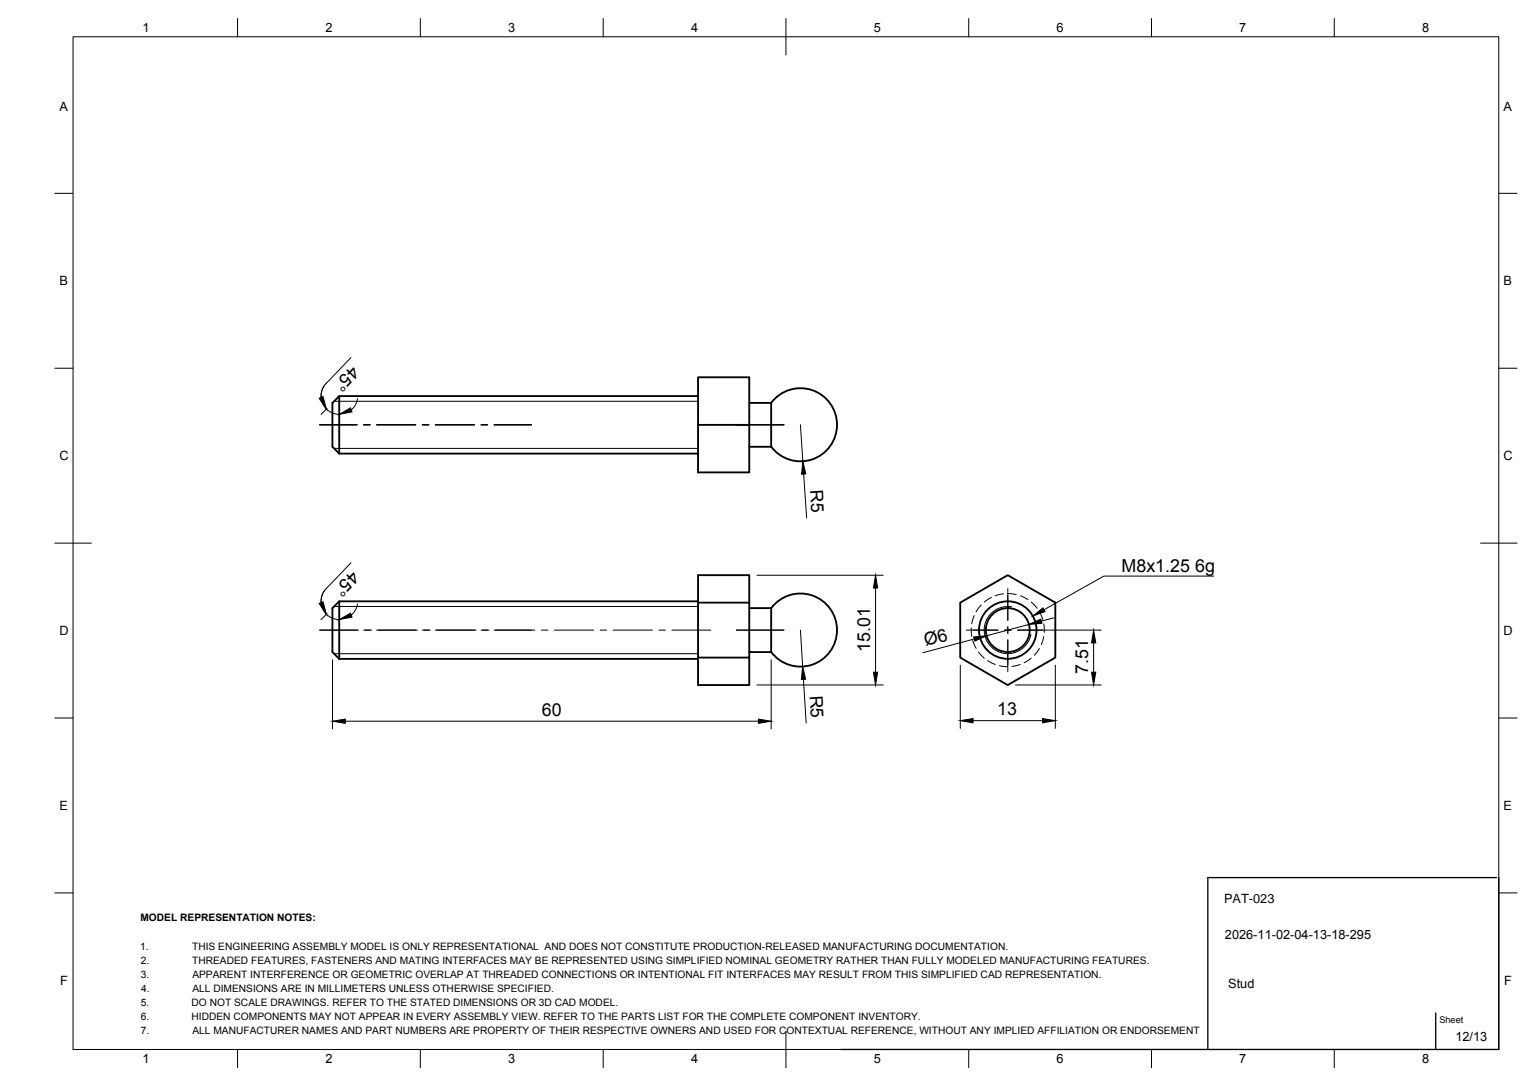
ISO-10303-21;
HEADER;
/* Generated by software containing ST-Developer
 * from STEP Tools, Inc. (www.steptools.com) 
 */

FILE_DESCRIPTION(
/* description */ ('PAT-023'),
/* implementation_level */ '2;1');

FILE_NAME(
/* name */ 'Stud.step',
/* time_stamp */ '2026-10-29T15:47:46-07:00',
/* author */ (''),
/* organization */ (''),
/* preprocessor_version */ 'ST-DEVELOPER v20.2',
/* originating_system */ 'Autodesk Translation Framework v15.17.0.0',
/* authorisation */ '');

FILE_SCHEMA (('AUTOMOTIVE_DESIGN { 1 0 10303 214 3 1 1 }'));
ENDSEC;

DATA;
#10=MECHANICAL_DESIGN_GEOMETRIC_PRESENTATION_REPRESENTATION('',(#89),#3773);
#62=SPHERICAL_SURFACE('',#2421,0.5);
#65=CONICAL_SURFACE('',#2418,0.35,0.78539816339745);
#73=SHAPE_REPRESENTATION_RELATIONSHIP('SRR','None',#3821,#81);
#81=ADVANCED_BREP_SHAPE_REPRESENTATION('',(#97),#3769);
#89=STYLED_ITEM('',(#3953),#97);
#97=MANIFOLD_SOLID_BREP('Body1',#2242);
#110=FACE_BOUND('',#395,.T.);
#111=FACE_BOUND('',#404,.T.);
#154=PLANE('',#2404);
#155=PLANE('',#2406);
#156=PLANE('',#2407);
#157=PLANE('',#2408);
#158=PLANE('',#2409);
#159=PLANE('',#2410);
#160=PLANE('',#2411);
#161=PLANE('',#2415);
#162=PLANE('',#2420);
#265=FACE_OUTER_BOUND('',#394,.T.);
#266=FACE_OUTER_BOUND('',#396,.T.);
#267=FACE_OUTER_BOUND('',#397,.T.);
#268=FACE_OUTER_BOUND('',#398,.T.);
#269=FACE_OUTER_BOUND('',#399,.T.);
#270=FACE_OUTER_BOUND('',#400,.T.);
#271=FACE_OUTER_BOUND('',#401,.T.);
#272=FACE_OUTER_BOUND('',#402,.T.);
#273=FACE_OUTER_BOUND('',#403,.T.);
#274=FACE_OUTER_BOUND('',#405,.T.);
#275=FACE_OUTER_BOUND('',#406,.T.);
#276=FACE_OUTER_BOUND('',#407,.T.);
#277=FACE_OUTER_BOUND('',#408,.T.);
#394=EDGE_LOOP('',(#1735,#1736,#1737,#1738,#1739,#1740));
#395=EDGE_LOOP('',(#1741));
#396=EDGE_LOOP('',(#1742,#1743,#1744,#1745));
#397=EDGE_LOOP('',(#1746,#1747,#1748,#1749));
#398=EDGE_LOOP('',(#1750,#1751,#1752,#1753));
#399=EDGE_LOOP('',(#1754,#1755,#1756,#1757));
#400=EDGE_LOOP('',(#1758,#1759,#1760,#1761));
#401=EDGE_LOOP('',(#1762,#1763,#1764,#1765));
#402=EDGE_LOOP('',(#1766,#1767,#1768,#1769));
#403=EDGE_LOOP('',(#1770,#1771,#1772,#1773,#1774,#1775));
#404=EDGE_LOOP('',(#1776));
#405=EDGE_LOOP('',(#1777,#1778,#1779,#1780));
#406=EDGE_LOOP('',(#1781,#1782,#1783,#1784));
#407=EDGE_LOOP('',(#1785));
#408=EDGE_LOOP('',(#1786,#1787,#1788));
#566=LINE('',#3342,#830);
#567=LINE('',#3344,#831);
#568=LINE('',#3346,#832);
#569=LINE('',#3348,#833);
#570=LINE('',#3350,#834);
#571=LINE('',#3351,#835);
#572=LINE('',#3357,#836);
#573=LINE('',#3358,#837);
#574=LINE('',#3359,#838);
#575=LINE('',#3362,#839);
#576=LINE('',#3363,#840);
#577=LINE('',#3366,#841);
#578=LINE('',#3367,#842);
#579=LINE('',#3370,#843);
#580=LINE('',#3371,#844);
#581=LINE('',#3374,#845);
#582=LINE('',#3375,#846);
#583=LINE('',#3377,#847);
#584=LINE('',#3382,#848);
#585=LINE('',#3388,#849);
#586=LINE('',#3392,#850);
#830=VECTOR('',#2739,1.);
#831=VECTOR('',#2740,1.);
#832=VECTOR('',#2741,1.);
#833=VECTOR('',#2742,1.);
#834=VECTOR('',#2743,1.);
#835=VECTOR('',#2744,1.);
#836=VECTOR('',#2749,1.);
#837=VECTOR('',#2750,1.);
#838=VECTOR('',#2751,1.);
#839=VECTOR('',#2754,1.);
#840=VECTOR('',#2755,1.);
#841=VECTOR('',#2758,1.);
#842=VECTOR('',#2759,1.);
#843=VECTOR('',#2762,1.);
#844=VECTOR('',#2763,1.);
#845=VECTOR('',#2766,1.);
#846=VECTOR('',#2767,1.);
#847=VECTOR('',#2770,1.);
#848=VECTOR('',#2775,0.3);
#849=VECTOR('',#2784,0.4);
#850=VECTOR('',#2789,0.35);
#1013=CIRCLE('',#2405,0.3933);
#1014=CIRCLE('',#2413,0.3);
#1015=CIRCLE('',#2414,0.3);
#1016=CIRCLE('',#2417,0.3933);
#1017=CIRCLE('',#2419,0.3);
#1018=CIRCLE('',#2422,0.5);
#1097=VERTEX_POINT('',#3340);
#1098=VERTEX_POINT('',#3341);
#1099=VERTEX_POINT('',#3343);
#1100=VERTEX_POINT('',#3345);
#1101=VERTEX_POINT('',#3347);
#1102=VERTEX_POINT('',#3349);
#1103=VERTEX_POINT('',#3352);
#1104=VERTEX_POINT('',#3355);
#1105=VERTEX_POINT('',#3356);
#1106=VERTEX_POINT('',#3361);
#1107=VERTEX_POINT('',#3365);
#1108=VERTEX_POINT('',#3369);
#1109=VERTEX_POINT('',#3373);
#1110=VERTEX_POINT('',#3379);
#1111=VERTEX_POINT('',#3381);
#1112=VERTEX_POINT('',#3386);
#1113=VERTEX_POINT('',#3390);
#1114=VERTEX_POINT('',#3395);
#1330=EDGE_CURVE('',#1097,#1098,#566,.T.);
#1331=EDGE_CURVE('',#1098,#1099,#567,.T.);
#1332=EDGE_CURVE('',#1099,#1100,#568,.T.);
#1333=EDGE_CURVE('',#1100,#1101,#569,.T.);
#1334=EDGE_CURVE('',#1101,#1102,#570,.T.);
#1335=EDGE_CURVE('',#1102,#1097,#571,.T.);
#1336=EDGE_CURVE('',#1103,#1103,#1013,.F.);
#1337=EDGE_CURVE('',#1104,#1105,#572,.T.);
#1338=EDGE_CURVE('',#1105,#1097,#573,.T.);
#1339=EDGE_CURVE('',#1104,#1102,#574,.T.);
#1340=EDGE_CURVE('',#1106,#1104,#575,.T.);
#1341=EDGE_CURVE('',#1106,#1101,#576,.T.);
#1342=EDGE_CURVE('',#1107,#1106,#577,.T.);
#1343=EDGE_CURVE('',#1107,#1100,#578,.T.);
#1344=EDGE_CURVE('',#1108,#1107,#579,.T.);
#1345=EDGE_CURVE('',#1108,#1099,#580,.T.);
#1346=EDGE_CURVE('',#1109,#1108,#581,.T.);
#1347=EDGE_CURVE('',#1109,#1098,#582,.T.);
#1348=EDGE_CURVE('',#1105,#1109,#583,.T.);
#1349=EDGE_CURVE('',#1110,#1110,#1014,.T.);
#1350=EDGE_CURVE('',#1110,#1111,#584,.T.);
#1351=EDGE_CURVE('',#1111,#1111,#1015,.T.);
#1352=EDGE_CURVE('',#1112,#1112,#1016,.F.);
#1353=EDGE_CURVE('',#1112,#1103,#585,.T.);
#1354=EDGE_CURVE('',#1113,#1113,#1017,.T.);
#1355=EDGE_CURVE('',#1113,#1112,#586,.T.);
#1356=EDGE_CURVE('',#1111,#1114,#1018,.T.);
#1735=ORIENTED_EDGE('',*,*,#1330,.T.);
#1736=ORIENTED_EDGE('',*,*,#1331,.T.);
#1737=ORIENTED_EDGE('',*,*,#1332,.T.);
#1738=ORIENTED_EDGE('',*,*,#1333,.T.);
#1739=ORIENTED_EDGE('',*,*,#1334,.T.);
#1740=ORIENTED_EDGE('',*,*,#1335,.T.);
#1741=ORIENTED_EDGE('',*,*,#1336,.F.);
#1742=ORIENTED_EDGE('',*,*,#1337,.T.);
#1743=ORIENTED_EDGE('',*,*,#1338,.T.);
#1744=ORIENTED_EDGE('',*,*,#1335,.F.);
#1745=ORIENTED_EDGE('',*,*,#1339,.F.);
#1746=ORIENTED_EDGE('',*,*,#1340,.T.);
#1747=ORIENTED_EDGE('',*,*,#1339,.T.);
#1748=ORIENTED_EDGE('',*,*,#1334,.F.);
#1749=ORIENTED_EDGE('',*,*,#1341,.F.);
#1750=ORIENTED_EDGE('',*,*,#1342,.T.);
#1751=ORIENTED_EDGE('',*,*,#1341,.T.);
#1752=ORIENTED_EDGE('',*,*,#1333,.F.);
#1753=ORIENTED_EDGE('',*,*,#1343,.F.);
#1754=ORIENTED_EDGE('',*,*,#1344,.T.);
#1755=ORIENTED_EDGE('',*,*,#1343,.T.);
#1756=ORIENTED_EDGE('',*,*,#1332,.F.);
#1757=ORIENTED_EDGE('',*,*,#1345,.F.);
#1758=ORIENTED_EDGE('',*,*,#1346,.T.);
#1759=ORIENTED_EDGE('',*,*,#1345,.T.);
#1760=ORIENTED_EDGE('',*,*,#1331,.F.);
#1761=ORIENTED_EDGE('',*,*,#1347,.F.);
#1762=ORIENTED_EDGE('',*,*,#1348,.T.);
#1763=ORIENTED_EDGE('',*,*,#1347,.T.);
#1764=ORIENTED_EDGE('',*,*,#1330,.F.);
#1765=ORIENTED_EDGE('',*,*,#1338,.F.);
#1766=ORIENTED_EDGE('',*,*,#1349,.F.);
#1767=ORIENTED_EDGE('',*,*,#1350,.T.);
#1768=ORIENTED_EDGE('',*,*,#1351,.F.);
#1769=ORIENTED_EDGE('',*,*,#1350,.F.);
#1770=ORIENTED_EDGE('',*,*,#1348,.F.);
#1771=ORIENTED_EDGE('',*,*,#1337,.F.);
#1772=ORIENTED_EDGE('',*,*,#1340,.F.);
#1773=ORIENTED_EDGE('',*,*,#1342,.F.);
#1774=ORIENTED_EDGE('',*,*,#1344,.F.);
#1775=ORIENTED_EDGE('',*,*,#1346,.F.);
#1776=ORIENTED_EDGE('',*,*,#1349,.T.);
#1777=ORIENTED_EDGE('',*,*,#1352,.F.);
#1778=ORIENTED_EDGE('',*,*,#1353,.T.);
#1779=ORIENTED_EDGE('',*,*,#1336,.T.);
#1780=ORIENTED_EDGE('',*,*,#1353,.F.);
#1781=ORIENTED_EDGE('',*,*,#1354,.F.);
#1782=ORIENTED_EDGE('',*,*,#1355,.T.);
#1783=ORIENTED_EDGE('',*,*,#1352,.T.);
#1784=ORIENTED_EDGE('',*,*,#1355,.F.);
#1785=ORIENTED_EDGE('',*,*,#1354,.T.);
#1786=ORIENTED_EDGE('',*,*,#1351,.T.);
#1787=ORIENTED_EDGE('',*,*,#1356,.T.);
#1788=ORIENTED_EDGE('',*,*,#1356,.F.);
#2114=CYLINDRICAL_SURFACE('',#2412,0.3);
#2115=CYLINDRICAL_SURFACE('',#2416,0.3933);
#2165=ADVANCED_FACE('',(#265,#110),#154,.T.);
#2166=ADVANCED_FACE('',(#266),#155,.T.);
#2167=ADVANCED_FACE('',(#267),#156,.T.);
#2168=ADVANCED_FACE('',(#268),#157,.T.);
#2169=ADVANCED_FACE('',(#269),#158,.T.);
#2170=ADVANCED_FACE('',(#270),#159,.T.);
#2171=ADVANCED_FACE('',(#271),#160,.T.);
#2172=ADVANCED_FACE('',(#272),#2114,.T.);
#2173=ADVANCED_FACE('',(#273,#111),#161,.T.);
#2174=ADVANCED_FACE('',(#274),#2115,.T.);
#2175=ADVANCED_FACE('',(#275),#65,.T.);
#2176=ADVANCED_FACE('',(#276),#162,.T.);
#2177=ADVANCED_FACE('',(#277),#62,.T.);
#2242=CLOSED_SHELL('',(#2165,#2166,#2167,#2168,#2169,#2170,#2171,#2172,
#2173,#2174,#2175,#2176,#2177));
#2403=AXIS2_PLACEMENT_3D('',#3338,#2735,#2736);
#2404=AXIS2_PLACEMENT_3D('',#3339,#2737,#2738);
#2405=AXIS2_PLACEMENT_3D('',#3353,#2745,#2746);
#2406=AXIS2_PLACEMENT_3D('',#3354,#2747,#2748);
#2407=AXIS2_PLACEMENT_3D('',#3360,#2752,#2753);
#2408=AXIS2_PLACEMENT_3D('',#3364,#2756,#2757);
#2409=AXIS2_PLACEMENT_3D('',#3368,#2760,#2761);
#2410=AXIS2_PLACEMENT_3D('',#3372,#2764,#2765);
#2411=AXIS2_PLACEMENT_3D('',#3376,#2768,#2769);
#2412=AXIS2_PLACEMENT_3D('',#3378,#2771,#2772);
#2413=AXIS2_PLACEMENT_3D('',#3380,#2773,#2774);
#2414=AXIS2_PLACEMENT_3D('',#3383,#2776,#2777);
#2415=AXIS2_PLACEMENT_3D('',#3384,#2778,#2779);
#2416=AXIS2_PLACEMENT_3D('',#3385,#2780,#2781);
#2417=AXIS2_PLACEMENT_3D('',#3387,#2782,#2783);
#2418=AXIS2_PLACEMENT_3D('',#3389,#2785,#2786);
#2419=AXIS2_PLACEMENT_3D('',#3391,#2787,#2788);
#2420=AXIS2_PLACEMENT_3D('',#3393,#2790,#2791);
#2421=AXIS2_PLACEMENT_3D('',#3394,#2792,#2793);
#2422=AXIS2_PLACEMENT_3D('',#3396,#2794,#2795);
#2735=DIRECTION('axis',(0.,0.,1.));
#2736=DIRECTION('refdir',(1.,0.,0.));
#2737=DIRECTION('center_axis',(0.,0.,1.));
#2738=DIRECTION('ref_axis',(1.,0.,0.));
#2739=DIRECTION('',(0.5,0.866025403784439,0.));
#2740=DIRECTION('',(-0.5,0.866025403784439,0.));
#2741=DIRECTION('',(-1.,1.4792020664489E-16,0.));
#2742=DIRECTION('',(-0.5,-0.866025403784439,0.));
#2743=DIRECTION('',(0.5,-0.866025403784439,0.));
#2744=DIRECTION('',(1.,-2.95840413289779E-16,0.));
#2745=DIRECTION('center_axis',(0.,0.,-1.));
#2746=DIRECTION('ref_axis',(1.,0.,0.));
#2747=DIRECTION('center_axis',(-2.95840413289779E-16,-1.,0.));
#2748=DIRECTION('ref_axis',(1.,-2.95840413289779E-16,0.));
#2749=DIRECTION('',(1.,-2.95840413289779E-16,0.));
#2750=DIRECTION('',(0.,0.,1.));
#2751=DIRECTION('',(0.,0.,1.));
#2752=DIRECTION('center_axis',(-0.866025403784439,-0.5,0.));
#2753=DIRECTION('ref_axis',(0.5,-0.866025403784439,0.));
#2754=DIRECTION('',(0.5,-0.866025403784439,0.));
#2755=DIRECTION('',(0.,0.,1.));
#2756=DIRECTION('center_axis',(-0.866025403784439,0.5,0.));
#2757=DIRECTION('ref_axis',(-0.5,-0.866025403784439,0.));
#2758=DIRECTION('',(-0.5,-0.866025403784439,0.));
#2759=DIRECTION('',(0.,0.,1.));
#2760=DIRECTION('center_axis',(1.4792020664489E-16,1.,0.));
#2761=DIRECTION('ref_axis',(-1.,1.4792020664489E-16,0.));
#2762=DIRECTION('',(-1.,1.4792020664489E-16,0.));
#2763=DIRECTION('',(0.,0.,1.));
#2764=DIRECTION('center_axis',(0.866025403784439,0.5,0.));
#2765=DIRECTION('ref_axis',(-0.5,0.866025403784439,0.));
#2766=DIRECTION('',(-0.5,0.866025403784439,0.));
#2767=DIRECTION('',(0.,0.,1.));
#2768=DIRECTION('center_axis',(0.866025403784439,-0.5,0.));
#2769=DIRECTION('ref_axis',(0.5,0.866025403784439,0.));
#2770=DIRECTION('',(0.5,0.866025403784439,0.));
#2771=DIRECTION('center_axis',(0.,0.,1.));
#2772=DIRECTION('ref_axis',(1.,0.,0.));
#2773=DIRECTION('center_axis',(0.,0.,1.));
#2774=DIRECTION('ref_axis',(1.,0.,0.));
#2775=DIRECTION('',(0.,0.,-1.));
#2776=DIRECTION('center_axis',(0.,0.,-1.));
#2777=DIRECTION('ref_axis',(1.,0.,0.));
#2778=DIRECTION('center_axis',(0.,0.,-1.));
#2779=DIRECTION('ref_axis',(-1.,0.,0.));
#2780=DIRECTION('center_axis',(0.,0.,1.));
#2781=DIRECTION('ref_axis',(1.,0.,0.));
#2782=DIRECTION('center_axis',(0.,0.,-1.));
#2783=DIRECTION('ref_axis',(1.,0.,0.));
#2784=DIRECTION('',(0.,0.,-1.));
#2785=DIRECTION('center_axis',(0.,0.,-1.));
#2786=DIRECTION('ref_axis',(1.,0.,0.));
#2787=DIRECTION('center_axis',(0.,0.,1.));
#2788=DIRECTION('ref_axis',(1.,0.,0.));
#2789=DIRECTION('',(-0.707106781186549,-8.65956056235495E-17,-0.707106781186546));
#2790=DIRECTION('center_axis',(0.,0.,1.));
#2791=DIRECTION('ref_axis',(1.,0.,0.));
#2792=DIRECTION('center_axis',(6.12323399573677E-17,0.,1.));
#2793=DIRECTION('ref_axis',(1.,0.,0.));
#2794=DIRECTION('center_axis',(1.22464679914735E-16,-1.,0.));
#2795=DIRECTION('ref_axis',(-1.,-1.22464679914735E-16,0.));
#3338=CARTESIAN_POINT('',(0.,0.,0.));
#3339=CARTESIAN_POINT('Origin',(0.,1.11022302462516E-16,2.5));
#3340=CARTESIAN_POINT('',(0.375277674973257,-0.65,2.5));
#3341=CARTESIAN_POINT('',(0.750555349946514,0.,2.5));
#3342=CARTESIAN_POINT('',(0.375277674973257,-0.65,2.5));
#3343=CARTESIAN_POINT('',(0.375277674973257,0.65,2.5));
#3344=CARTESIAN_POINT('',(0.750555349946514,0.,2.5));
#3345=CARTESIAN_POINT('',(-0.375277674973257,0.65,2.5));
#3346=CARTESIAN_POINT('',(0.375277674973257,0.65,2.5));
#3347=CARTESIAN_POINT('',(-0.750555349946514,1.11022302462516E-16,2.5));
#3348=CARTESIAN_POINT('',(-0.375277674973257,0.65,2.5));
#3349=CARTESIAN_POINT('',(-0.375277674973257,-0.65,2.5));
#3350=CARTESIAN_POINT('',(-0.750555349946514,9.19165206894919E-17,2.5));
#3351=CARTESIAN_POINT('',(-0.375277674973257,-0.65,2.5));
#3352=CARTESIAN_POINT('',(-0.3933,4.81653586104654E-17,2.5));
#3353=CARTESIAN_POINT('Origin',(0.,0.,2.5));
#3354=CARTESIAN_POINT('Origin',(-0.375277674973257,-0.65,1.8));
#3355=CARTESIAN_POINT('',(-0.375277674973257,-0.65,1.8));
#3356=CARTESIAN_POINT('',(0.375277674973257,-0.65,1.8));
#3357=CARTESIAN_POINT('',(-0.375277674973257,-0.65,1.8));
#3358=CARTESIAN_POINT('',(0.375277674973257,-0.65,1.8));
#3359=CARTESIAN_POINT('',(-0.375277674973257,-0.65,1.8));
#3360=CARTESIAN_POINT('Origin',(-0.750555349946514,9.19165206894919E-17,
1.8));
#3361=CARTESIAN_POINT('',(-0.750555349946514,9.19165206894919E-17,1.8));
#3362=CARTESIAN_POINT('',(-0.750555349946514,9.19165206894919E-17,1.8));
#3363=CARTESIAN_POINT('',(-0.750555349946514,9.19165206894919E-17,1.8));
#3364=CARTESIAN_POINT('Origin',(-0.375277674973257,0.65,1.8));
#3365=CARTESIAN_POINT('',(-0.375277674973257,0.65,1.8));
#3366=CARTESIAN_POINT('',(-0.375277674973257,0.65,1.8));
#3367=CARTESIAN_POINT('',(-0.375277674973257,0.65,1.8));
#3368=CARTESIAN_POINT('Origin',(0.375277674973257,0.65,1.8));
#3369=CARTESIAN_POINT('',(0.375277674973257,0.65,1.8));
#3370=CARTESIAN_POINT('',(0.375277674973257,0.65,1.8));
#3371=CARTESIAN_POINT('',(0.375277674973257,0.65,1.8));
#3372=CARTESIAN_POINT('Origin',(0.750555349946514,0.,1.8));
#3373=CARTESIAN_POINT('',(0.750555349946514,0.,1.8));
#3374=CARTESIAN_POINT('',(0.750555349946514,0.,1.8));
#3375=CARTESIAN_POINT('',(0.750555349946514,0.,1.8));
#3376=CARTESIAN_POINT('Origin',(0.375277674973257,-0.65,1.8));
#3377=CARTESIAN_POINT('',(0.375277674973257,-0.65,1.8));
#3378=CARTESIAN_POINT('Origin',(0.,0.,1.45));
#3379=CARTESIAN_POINT('',(-0.3,-3.67394039744206E-17,1.8));
#3380=CARTESIAN_POINT('Origin',(0.,0.,1.8));
#3381=CARTESIAN_POINT('',(-0.3,3.67394039744206E-17,1.5));
#3382=CARTESIAN_POINT('',(-0.3,-3.67394039744206E-17,1.45));
#3383=CARTESIAN_POINT('Origin',(0.,0.,1.5));
#3384=CARTESIAN_POINT('Origin',(0.4,0.,1.8));
#3385=CARTESIAN_POINT('Origin',(0.,0.,4.6));
#3386=CARTESIAN_POINT('',(-0.3933,4.81653586104654E-17,7.4067));
#3387=CARTESIAN_POINT('Origin',(0.,0.,7.4067));
#3388=CARTESIAN_POINT('',(-0.3933,-4.81653586104654E-17,4.6));
#3389=CARTESIAN_POINT('Origin',(0.,0.,7.45));
#3390=CARTESIAN_POINT('',(-0.3,-3.67394039744206E-17,7.5));
#3391=CARTESIAN_POINT('Origin',(0.,0.,7.5));
#3392=CARTESIAN_POINT('',(-0.35,-4.28626379701574E-17,7.45));
#3393=CARTESIAN_POINT('Origin',(0.,0.,7.5));
#3394=CARTESIAN_POINT('Origin',(-5.55111512312578E-17,0.,1.1));
#3395=CARTESIAN_POINT('',(-8.61273212099417E-17,-3.74939945665464E-33,0.6));
#3396=CARTESIAN_POINT('Origin',(-5.55111512312578E-17,0.,1.1));
#3756=UNCERTAINTY_MEASURE_WITH_UNIT(LENGTH_MEASURE(0.001),#3774,
'DISTANCE_ACCURACY_VALUE',
'Maximum model space distance between geometric entities at asserted c
onnectivities');
#3760=UNCERTAINTY_MEASURE_WITH_UNIT(LENGTH_MEASURE(0.001),#3774,
'DISTANCE_ACCURACY_VALUE',
'Maximum model space distance between geometric entities at asserted c
onnectivities');
#3769=(
GEOMETRIC_REPRESENTATION_CONTEXT(3)
GLOBAL_UNCERTAINTY_ASSIGNED_CONTEXT((#3756))
GLOBAL_UNIT_ASSIGNED_CONTEXT((#3774,#3776,#3777))
REPRESENTATION_CONTEXT('','3D')
);
#3773=(
GEOMETRIC_REPRESENTATION_CONTEXT(3)
GLOBAL_UNCERTAINTY_ASSIGNED_CONTEXT((#3760))
GLOBAL_UNIT_ASSIGNED_CONTEXT((#3774,#3776,#3777))
REPRESENTATION_CONTEXT('','3D')
);
#3774=(
LENGTH_UNIT()
NAMED_UNIT(*)
SI_UNIT(.CENTI.,.METRE.)
);
#3776=(
NAMED_UNIT(*)
PLANE_ANGLE_UNIT()
SI_UNIT($,.RADIAN.)
);
#3777=(
NAMED_UNIT(*)
SI_UNIT($,.STERADIAN.)
SOLID_ANGLE_UNIT()
);
#3786=SHAPE_DEFINITION_REPRESENTATION(#3798,#3821);
#3798=PRODUCT_DEFINITION_SHAPE('',$,#3834);
#3821=SHAPE_REPRESENTATION('',(#2403),#3769);
#3825=PRODUCT_DEFINITION_CONTEXT('part definition',#3863,'design');
#3834=PRODUCT_DEFINITION('Stud','Stud',#3846,#3825);
#3846=PRODUCT_DEFINITION_FORMATION('',$,#3873);
#3863=APPLICATION_CONTEXT(
'Core Data for Automotive Mechanical Design Process');
#3864=PRODUCT_CONTEXT('part definition',#3863,'mechanical');
#3873=PRODUCT('Stud','Stud','Stud',(#3864));
#3947=COLOUR_RGB('Black',0.12,0.14,0.17);
#3948=FILL_AREA_STYLE_COLOUR('',#3947);
#3949=FILL_AREA_STYLE('',(#3948));
#3950=SURFACE_STYLE_FILL_AREA(#3949);
#3951=SURFACE_SIDE_STYLE('',(#3950));
#3952=SURFACE_STYLE_USAGE(.BOTH.,#3951);
#3953=PRESENTATION_STYLE_ASSIGNMENT((#3952));
ENDSEC;
END-ISO-10303-21;
